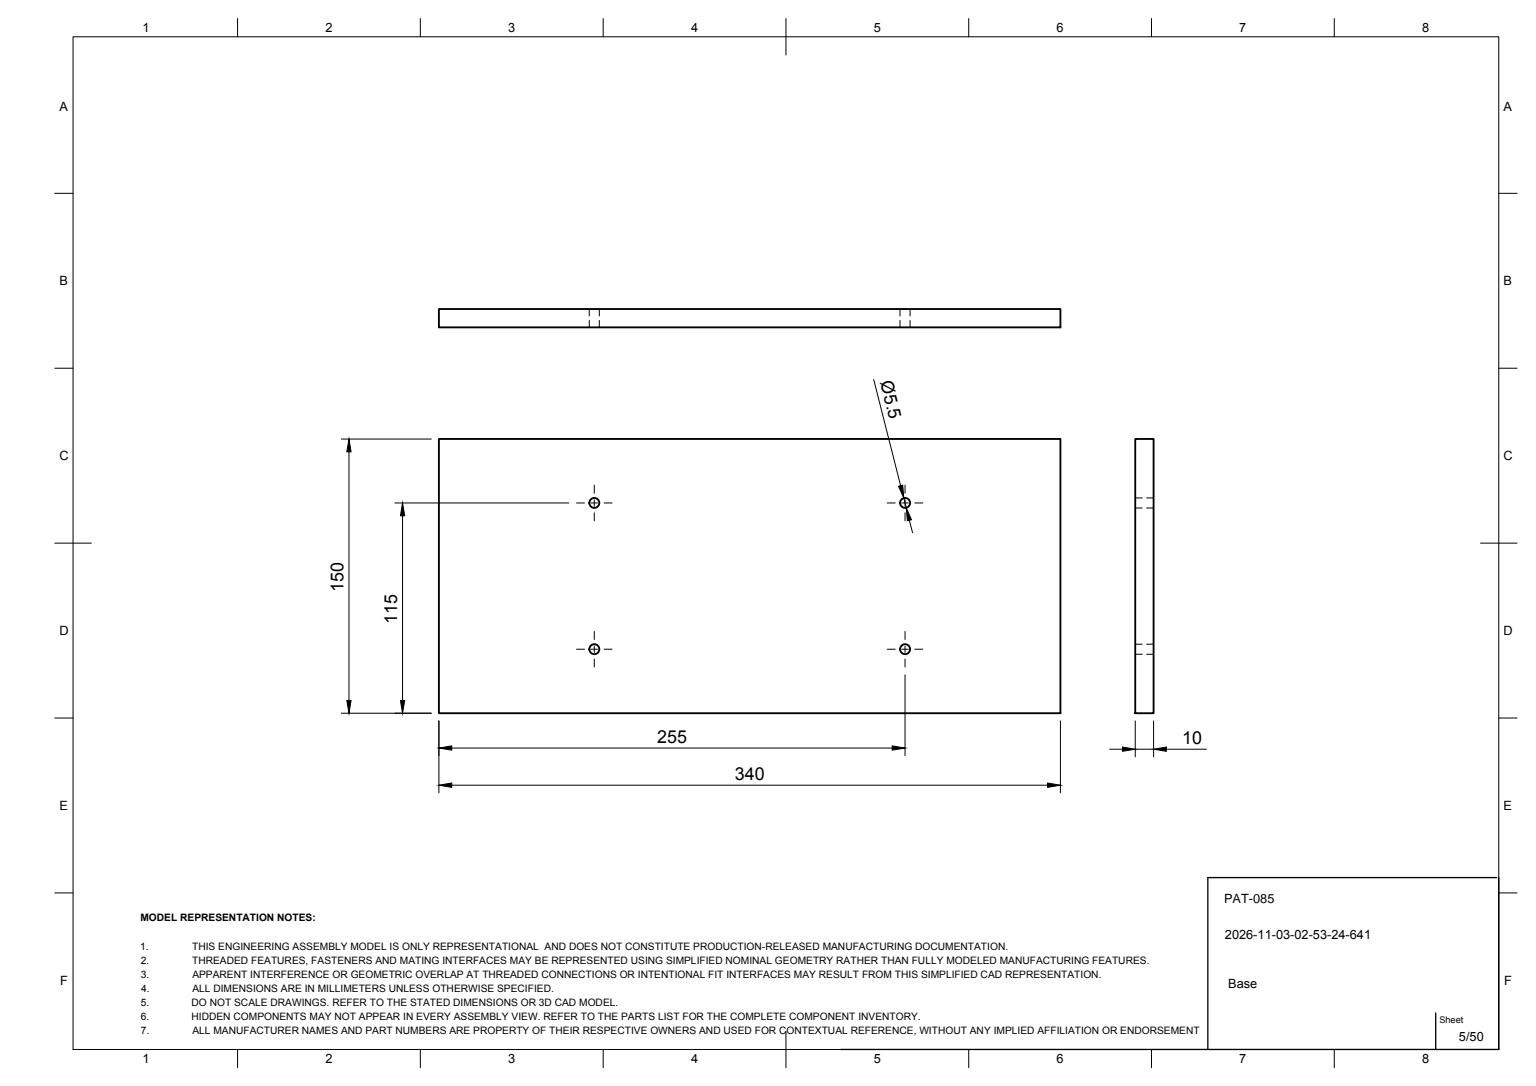
ISO-10303-21;
HEADER;
/* Generated by software containing ST-Developer
 * from STEP Tools, Inc. (www.steptools.com) 
 */

FILE_DESCRIPTION(
/* description */ ('Rack and pinion manual slide'),
/* implementation_level */ '2;1');

FILE_NAME(
/* name */ 'Base.step',
/* time_stamp */ '2026-10-28T03:22:49-07:00',
/* author */ (''),
/* organization */ (''),
/* preprocessor_version */ 'ST-DEVELOPER v20.2',
/* originating_system */ 'Autodesk Translation Framework v15.17.0.0',
/* authorisation */ '');

FILE_SCHEMA (('AUTOMOTIVE_DESIGN { 1 0 10303 214 3 1 1 }'));
ENDSEC;

DATA;
#10=MECHANICAL_DESIGN_GEOMETRIC_PRESENTATION_REPRESENTATION('',(#732),#34851);
#640=SHAPE_REPRESENTATION_RELATIONSHIP('SRR','None',#35075,#686);
#686=ADVANCED_BREP_SHAPE_REPRESENTATION('',(#785),#34800);
#732=STYLED_ITEM('',(#35390),#785);
#785=MANIFOLD_SOLID_BREP('Body1',#13752);
#833=FACE_BOUND('',#2283,.T.);
#834=FACE_BOUND('',#2284,.T.);
#835=FACE_BOUND('',#2285,.T.);
#836=FACE_BOUND('',#2286,.T.);
#837=FACE_BOUND('',#2288,.T.);
#838=FACE_BOUND('',#2289,.T.);
#839=FACE_BOUND('',#2290,.T.);
#840=FACE_BOUND('',#2291,.T.);
#1044=PLANE('',#14332);
#1045=PLANE('',#14333);
#1046=PLANE('',#14334);
#1047=PLANE('',#14335);
#1048=PLANE('',#14336);
#1049=PLANE('',#14337);
#1535=FACE_OUTER_BOUND('',#2274,.T.);
#1536=FACE_OUTER_BOUND('',#2275,.T.);
#1537=FACE_OUTER_BOUND('',#2276,.T.);
#1538=FACE_OUTER_BOUND('',#2277,.T.);
#1539=FACE_OUTER_BOUND('',#2278,.T.);
#1540=FACE_OUTER_BOUND('',#2279,.T.);
#1541=FACE_OUTER_BOUND('',#2280,.T.);
#1542=FACE_OUTER_BOUND('',#2281,.T.);
#1543=FACE_OUTER_BOUND('',#2282,.T.);
#1544=FACE_OUTER_BOUND('',#2287,.T.);
#2274=EDGE_LOOP('',(#9234,#9235,#9236,#9237));
#2275=EDGE_LOOP('',(#9238,#9239,#9240,#9241));
#2276=EDGE_LOOP('',(#9242,#9243,#9244,#9245));
#2277=EDGE_LOOP('',(#9246,#9247,#9248,#9249));
#2278=EDGE_LOOP('',(#9250,#9251,#9252,#9253));
#2279=EDGE_LOOP('',(#9254,#9255,#9256,#9257));
#2280=EDGE_LOOP('',(#9258,#9259,#9260,#9261));
#2281=EDGE_LOOP('',(#9262,#9263,#9264,#9265));
#2282=EDGE_LOOP('',(#9266,#9267,#9268,#9269));
#2283=EDGE_LOOP('',(#9270));
#2284=EDGE_LOOP('',(#9271));
#2285=EDGE_LOOP('',(#9272));
#2286=EDGE_LOOP('',(#9273));
#2287=EDGE_LOOP('',(#9274,#9275,#9276,#9277));
#2288=EDGE_LOOP('',(#9278));
#2289=EDGE_LOOP('',(#9279));
#2290=EDGE_LOOP('',(#9280));
#2291=EDGE_LOOP('',(#9281));
#3224=LINE('',#19464,#4515);
#3225=LINE('',#19470,#4516);
#3226=LINE('',#19476,#4517);
#3227=LINE('',#19482,#4518);
#3228=LINE('',#19487,#4519);
#3229=LINE('',#19489,#4520);
#3230=LINE('',#19491,#4521);
#3231=LINE('',#19492,#4522);
#3232=LINE('',#19495,#4523);
#3233=LINE('',#19497,#4524);
#3234=LINE('',#19498,#4525);
#3235=LINE('',#19501,#4526);
#3236=LINE('',#19503,#4527);
#3237=LINE('',#19504,#4528);
#3238=LINE('',#19506,#4529);
#3239=LINE('',#19507,#4530);
#4515=VECTOR('',#15610,0.274999999999999);
#4516=VECTOR('',#15617,0.274999999999999);
#4517=VECTOR('',#15624,0.275);
#4518=VECTOR('',#15631,0.275);
#4519=VECTOR('',#15636,1.);
#4520=VECTOR('',#15637,1.);
#4521=VECTOR('',#15638,1.);
#4522=VECTOR('',#15639,1.);
#4523=VECTOR('',#15642,1.);
#4524=VECTOR('',#15643,1.);
#4525=VECTOR('',#15644,1.);
#4526=VECTOR('',#15647,1.);
#4527=VECTOR('',#15648,1.);
#4528=VECTOR('',#15649,1.);
#4529=VECTOR('',#15652,1.);
#4530=VECTOR('',#15653,1.);
#5806=CIRCLE('',#14321,0.274999999999999);
#5807=CIRCLE('',#14322,0.274999999999999);
#5808=CIRCLE('',#14324,0.274999999999999);
#5809=CIRCLE('',#14325,0.274999999999999);
#5810=CIRCLE('',#14327,0.275);
#5811=CIRCLE('',#14328,0.275);
#5812=CIRCLE('',#14330,0.275);
#5813=CIRCLE('',#14331,0.275);
#6224=VERTEX_POINT('',#19461);
#6225=VERTEX_POINT('',#19463);
#6226=VERTEX_POINT('',#19467);
#6227=VERTEX_POINT('',#19469);
#6228=VERTEX_POINT('',#19473);
#6229=VERTEX_POINT('',#19475);
#6230=VERTEX_POINT('',#19479);
#6231=VERTEX_POINT('',#19481);
#6232=VERTEX_POINT('',#19485);
#6233=VERTEX_POINT('',#19486);
#6234=VERTEX_POINT('',#19488);
#6235=VERTEX_POINT('',#19490);
#6236=VERTEX_POINT('',#19494);
#6237=VERTEX_POINT('',#19496);
#6238=VERTEX_POINT('',#19500);
#6239=VERTEX_POINT('',#19502);
#7429=EDGE_CURVE('',#6224,#6224,#5806,.T.);
#7430=EDGE_CURVE('',#6224,#6225,#3224,.T.);
#7431=EDGE_CURVE('',#6225,#6225,#5807,.T.);
#7432=EDGE_CURVE('',#6226,#6226,#5808,.T.);
#7433=EDGE_CURVE('',#6226,#6227,#3225,.T.);
#7434=EDGE_CURVE('',#6227,#6227,#5809,.T.);
#7435=EDGE_CURVE('',#6228,#6228,#5810,.T.);
#7436=EDGE_CURVE('',#6228,#6229,#3226,.T.);
#7437=EDGE_CURVE('',#6229,#6229,#5811,.T.);
#7438=EDGE_CURVE('',#6230,#6230,#5812,.T.);
#7439=EDGE_CURVE('',#6230,#6231,#3227,.T.);
#7440=EDGE_CURVE('',#6231,#6231,#5813,.T.);
#7441=EDGE_CURVE('',#6232,#6233,#3228,.T.);
#7442=EDGE_CURVE('',#6233,#6234,#3229,.T.);
#7443=EDGE_CURVE('',#6235,#6234,#3230,.T.);
#7444=EDGE_CURVE('',#6232,#6235,#3231,.T.);
#7445=EDGE_CURVE('',#6236,#6232,#3232,.T.);
#7446=EDGE_CURVE('',#6237,#6235,#3233,.T.);
#7447=EDGE_CURVE('',#6236,#6237,#3234,.T.);
#7448=EDGE_CURVE('',#6238,#6236,#3235,.T.);
#7449=EDGE_CURVE('',#6239,#6237,#3236,.T.);
#7450=EDGE_CURVE('',#6238,#6239,#3237,.T.);
#7451=EDGE_CURVE('',#6233,#6238,#3238,.T.);
#7452=EDGE_CURVE('',#6234,#6239,#3239,.T.);
#9234=ORIENTED_EDGE('',*,*,#7429,.F.);
#9235=ORIENTED_EDGE('',*,*,#7430,.T.);
#9236=ORIENTED_EDGE('',*,*,#7431,.F.);
#9237=ORIENTED_EDGE('',*,*,#7430,.F.);
#9238=ORIENTED_EDGE('',*,*,#7432,.F.);
#9239=ORIENTED_EDGE('',*,*,#7433,.T.);
#9240=ORIENTED_EDGE('',*,*,#7434,.F.);
#9241=ORIENTED_EDGE('',*,*,#7433,.F.);
#9242=ORIENTED_EDGE('',*,*,#7435,.F.);
#9243=ORIENTED_EDGE('',*,*,#7436,.T.);
#9244=ORIENTED_EDGE('',*,*,#7437,.F.);
#9245=ORIENTED_EDGE('',*,*,#7436,.F.);
#9246=ORIENTED_EDGE('',*,*,#7438,.F.);
#9247=ORIENTED_EDGE('',*,*,#7439,.T.);
#9248=ORIENTED_EDGE('',*,*,#7440,.F.);
#9249=ORIENTED_EDGE('',*,*,#7439,.F.);
#9250=ORIENTED_EDGE('',*,*,#7441,.T.);
#9251=ORIENTED_EDGE('',*,*,#7442,.T.);
#9252=ORIENTED_EDGE('',*,*,#7443,.F.);
#9253=ORIENTED_EDGE('',*,*,#7444,.F.);
#9254=ORIENTED_EDGE('',*,*,#7445,.T.);
#9255=ORIENTED_EDGE('',*,*,#7444,.T.);
#9256=ORIENTED_EDGE('',*,*,#7446,.F.);
#9257=ORIENTED_EDGE('',*,*,#7447,.F.);
#9258=ORIENTED_EDGE('',*,*,#7448,.T.);
#9259=ORIENTED_EDGE('',*,*,#7447,.T.);
#9260=ORIENTED_EDGE('',*,*,#7449,.F.);
#9261=ORIENTED_EDGE('',*,*,#7450,.F.);
#9262=ORIENTED_EDGE('',*,*,#7451,.T.);
#9263=ORIENTED_EDGE('',*,*,#7450,.T.);
#9264=ORIENTED_EDGE('',*,*,#7452,.F.);
#9265=ORIENTED_EDGE('',*,*,#7442,.F.);
#9266=ORIENTED_EDGE('',*,*,#7452,.T.);
#9267=ORIENTED_EDGE('',*,*,#7449,.T.);
#9268=ORIENTED_EDGE('',*,*,#7446,.T.);
#9269=ORIENTED_EDGE('',*,*,#7443,.T.);
#9270=ORIENTED_EDGE('',*,*,#7431,.T.);
#9271=ORIENTED_EDGE('',*,*,#7434,.T.);
#9272=ORIENTED_EDGE('',*,*,#7437,.T.);
#9273=ORIENTED_EDGE('',*,*,#7440,.T.);
#9274=ORIENTED_EDGE('',*,*,#7451,.F.);
#9275=ORIENTED_EDGE('',*,*,#7441,.F.);
#9276=ORIENTED_EDGE('',*,*,#7445,.F.);
#9277=ORIENTED_EDGE('',*,*,#7448,.F.);
#9278=ORIENTED_EDGE('',*,*,#7429,.T.);
#9279=ORIENTED_EDGE('',*,*,#7432,.T.);
#9280=ORIENTED_EDGE('',*,*,#7435,.T.);
#9281=ORIENTED_EDGE('',*,*,#7438,.T.);
#12844=CYLINDRICAL_SURFACE('',#14320,0.274999999999999);
#12845=CYLINDRICAL_SURFACE('',#14323,0.274999999999999);
#12846=CYLINDRICAL_SURFACE('',#14326,0.275);
#12847=CYLINDRICAL_SURFACE('',#14329,0.275);
#13013=ADVANCED_FACE('',(#1535),#12844,.F.);
#13014=ADVANCED_FACE('',(#1536),#12845,.F.);
#13015=ADVANCED_FACE('',(#1537),#12846,.F.);
#13016=ADVANCED_FACE('',(#1538),#12847,.F.);
#13017=ADVANCED_FACE('',(#1539),#1044,.T.);
#13018=ADVANCED_FACE('',(#1540),#1045,.T.);
#13019=ADVANCED_FACE('',(#1541),#1046,.T.);
#13020=ADVANCED_FACE('',(#1542),#1047,.T.);
#13021=ADVANCED_FACE('',(#1543,#833,#834,#835,#836),#1048,.T.);
#13022=ADVANCED_FACE('',(#1544,#837,#838,#839,#840),#1049,.F.);
#13752=CLOSED_SHELL('',(#13013,#13014,#13015,#13016,#13017,#13018,#13019,
#13020,#13021,#13022));
#14319=AXIS2_PLACEMENT_3D('',#19459,#15604,#15605);
#14320=AXIS2_PLACEMENT_3D('',#19460,#15606,#15607);
#14321=AXIS2_PLACEMENT_3D('',#19462,#15608,#15609);
#14322=AXIS2_PLACEMENT_3D('',#19465,#15611,#15612);
#14323=AXIS2_PLACEMENT_3D('',#19466,#15613,#15614);
#14324=AXIS2_PLACEMENT_3D('',#19468,#15615,#15616);
#14325=AXIS2_PLACEMENT_3D('',#19471,#15618,#15619);
#14326=AXIS2_PLACEMENT_3D('',#19472,#15620,#15621);
#14327=AXIS2_PLACEMENT_3D('',#19474,#15622,#15623);
#14328=AXIS2_PLACEMENT_3D('',#19477,#15625,#15626);
#14329=AXIS2_PLACEMENT_3D('',#19478,#15627,#15628);
#14330=AXIS2_PLACEMENT_3D('',#19480,#15629,#15630);
#14331=AXIS2_PLACEMENT_3D('',#19483,#15632,#15633);
#14332=AXIS2_PLACEMENT_3D('',#19484,#15634,#15635);
#14333=AXIS2_PLACEMENT_3D('',#19493,#15640,#15641);
#14334=AXIS2_PLACEMENT_3D('',#19499,#15645,#15646);
#14335=AXIS2_PLACEMENT_3D('',#19505,#15650,#15651);
#14336=AXIS2_PLACEMENT_3D('',#19508,#15654,#15655);
#14337=AXIS2_PLACEMENT_3D('',#19509,#15656,#15657);
#15604=DIRECTION('axis',(0.,0.,1.));
#15605=DIRECTION('refdir',(1.,0.,0.));
#15606=DIRECTION('center_axis',(0.,0.,1.));
#15607=DIRECTION('ref_axis',(1.,0.,0.));
#15608=DIRECTION('center_axis',(0.,0.,1.));
#15609=DIRECTION('ref_axis',(1.,0.,0.));
#15610=DIRECTION('',(0.,0.,1.));
#15611=DIRECTION('center_axis',(0.,0.,-1.));
#15612=DIRECTION('ref_axis',(1.,0.,0.));
#15613=DIRECTION('center_axis',(0.,0.,1.));
#15614=DIRECTION('ref_axis',(1.,0.,0.));
#15615=DIRECTION('center_axis',(0.,0.,1.));
#15616=DIRECTION('ref_axis',(1.,0.,0.));
#15617=DIRECTION('',(0.,0.,1.));
#15618=DIRECTION('center_axis',(0.,0.,-1.));
#15619=DIRECTION('ref_axis',(1.,0.,0.));
#15620=DIRECTION('center_axis',(0.,0.,1.));
#15621=DIRECTION('ref_axis',(1.,0.,0.));
#15622=DIRECTION('center_axis',(0.,0.,1.));
#15623=DIRECTION('ref_axis',(1.,0.,0.));
#15624=DIRECTION('',(0.,0.,1.));
#15625=DIRECTION('center_axis',(0.,0.,-1.));
#15626=DIRECTION('ref_axis',(1.,0.,0.));
#15627=DIRECTION('center_axis',(0.,0.,1.));
#15628=DIRECTION('ref_axis',(1.,0.,0.));
#15629=DIRECTION('center_axis',(0.,0.,1.));
#15630=DIRECTION('ref_axis',(1.,0.,0.));
#15631=DIRECTION('',(0.,0.,1.));
#15632=DIRECTION('center_axis',(0.,0.,-1.));
#15633=DIRECTION('ref_axis',(1.,0.,0.));
#15634=DIRECTION('center_axis',(0.,1.,0.));
#15635=DIRECTION('ref_axis',(-1.,0.,0.));
#15636=DIRECTION('',(-1.,0.,0.));
#15637=DIRECTION('',(0.,0.,1.));
#15638=DIRECTION('',(-1.,0.,0.));
#15639=DIRECTION('',(0.,0.,1.));
#15640=DIRECTION('center_axis',(1.,0.,0.));
#15641=DIRECTION('ref_axis',(0.,1.,0.));
#15642=DIRECTION('',(0.,1.,0.));
#15643=DIRECTION('',(0.,1.,0.));
#15644=DIRECTION('',(0.,0.,1.));
#15645=DIRECTION('center_axis',(0.,-1.,0.));
#15646=DIRECTION('ref_axis',(1.,0.,0.));
#15647=DIRECTION('',(1.,0.,0.));
#15648=DIRECTION('',(1.,0.,0.));
#15649=DIRECTION('',(0.,0.,1.));
#15650=DIRECTION('center_axis',(-1.,0.,0.));
#15651=DIRECTION('ref_axis',(0.,-1.,0.));
#15652=DIRECTION('',(0.,-1.,0.));
#15653=DIRECTION('',(0.,-1.,0.));
#15654=DIRECTION('center_axis',(0.,0.,1.));
#15655=DIRECTION('ref_axis',(1.,0.,0.));
#15656=DIRECTION('center_axis',(0.,0.,1.));
#15657=DIRECTION('ref_axis',(1.,0.,0.));
#19459=CARTESIAN_POINT('',(0.,0.,0.));
#19460=CARTESIAN_POINT('Origin',(19.5,4.,-0.1));
#19461=CARTESIAN_POINT('',(19.225,4.,0.));
#19462=CARTESIAN_POINT('Origin',(19.5,4.,0.));
#19463=CARTESIAN_POINT('',(19.225,4.,1.));
#19464=CARTESIAN_POINT('',(19.225,4.,-0.1));
#19465=CARTESIAN_POINT('Origin',(19.5,4.,1.));
#19466=CARTESIAN_POINT('Origin',(19.5,-4.,-0.1));
#19467=CARTESIAN_POINT('',(19.225,-4.,0.));
#19468=CARTESIAN_POINT('Origin',(19.5,-4.,0.));
#19469=CARTESIAN_POINT('',(19.225,-4.,1.));
#19470=CARTESIAN_POINT('',(19.225,-4.,-0.1));
#19471=CARTESIAN_POINT('Origin',(19.5,-4.,1.));
#19472=CARTESIAN_POINT('Origin',(2.5,4.,-0.1));
#19473=CARTESIAN_POINT('',(2.225,4.,0.));
#19474=CARTESIAN_POINT('Origin',(2.5,4.,0.));
#19475=CARTESIAN_POINT('',(2.225,4.,1.));
#19476=CARTESIAN_POINT('',(2.225,4.,-0.1));
#19477=CARTESIAN_POINT('Origin',(2.5,4.,1.));
#19478=CARTESIAN_POINT('Origin',(2.5,-4.,-0.1));
#19479=CARTESIAN_POINT('',(2.225,-4.,0.));
#19480=CARTESIAN_POINT('Origin',(2.5,-4.,0.));
#19481=CARTESIAN_POINT('',(2.225,-4.,1.));
#19482=CARTESIAN_POINT('',(2.225,-4.,-0.1));
#19483=CARTESIAN_POINT('Origin',(2.5,-4.,1.));
#19484=CARTESIAN_POINT('Origin',(28.,7.5,0.));
#19485=CARTESIAN_POINT('',(28.,7.5,0.));
#19486=CARTESIAN_POINT('',(-6.,7.5,0.));
#19487=CARTESIAN_POINT('',(28.,7.5,0.));
#19488=CARTESIAN_POINT('',(-6.,7.5,1.));
#19489=CARTESIAN_POINT('',(-6.,7.5,0.));
#19490=CARTESIAN_POINT('',(28.,7.5,1.));
#19491=CARTESIAN_POINT('',(28.,7.5,1.));
#19492=CARTESIAN_POINT('',(28.,7.5,0.));
#19493=CARTESIAN_POINT('Origin',(28.,-7.5,0.));
#19494=CARTESIAN_POINT('',(28.,-7.5,0.));
#19495=CARTESIAN_POINT('',(28.,-7.5,0.));
#19496=CARTESIAN_POINT('',(28.,-7.5,1.));
#19497=CARTESIAN_POINT('',(28.,-7.5,1.));
#19498=CARTESIAN_POINT('',(28.,-7.5,0.));
#19499=CARTESIAN_POINT('Origin',(-6.,-7.5,0.));
#19500=CARTESIAN_POINT('',(-6.,-7.5,0.));
#19501=CARTESIAN_POINT('',(-6.,-7.5,0.));
#19502=CARTESIAN_POINT('',(-6.,-7.5,1.));
#19503=CARTESIAN_POINT('',(-6.,-7.5,1.));
#19504=CARTESIAN_POINT('',(-6.,-7.5,0.));
#19505=CARTESIAN_POINT('Origin',(-6.,7.5,0.));
#19506=CARTESIAN_POINT('',(-6.,7.5,0.));
#19507=CARTESIAN_POINT('',(-6.,7.5,1.));
#19508=CARTESIAN_POINT('Origin',(11.,0.,1.));
#19509=CARTESIAN_POINT('Origin',(11.,0.,0.));
#34746=UNCERTAINTY_MEASURE_WITH_UNIT(LENGTH_MEASURE(0.001),#34852,
'DISTANCE_ACCURACY_VALUE',
'Maximum model space distance between geometric entities at asserted c
onnectivities');
#34797=UNCERTAINTY_MEASURE_WITH_UNIT(LENGTH_MEASURE(0.001),#34852,
'DISTANCE_ACCURACY_VALUE',
'Maximum model space distance between geometric entities at asserted c
onnectivities');
#34800=(
GEOMETRIC_REPRESENTATION_CONTEXT(3)
GLOBAL_UNCERTAINTY_ASSIGNED_CONTEXT((#34746))
GLOBAL_UNIT_ASSIGNED_CONTEXT((#34852,#34854,#34855))
REPRESENTATION_CONTEXT('','3D')
);
#34851=(
GEOMETRIC_REPRESENTATION_CONTEXT(3)
GLOBAL_UNCERTAINTY_ASSIGNED_CONTEXT((#34797))
GLOBAL_UNIT_ASSIGNED_CONTEXT((#34852,#34854,#34855))
REPRESENTATION_CONTEXT('','3D')
);
#34852=(
LENGTH_UNIT()
NAMED_UNIT(*)
SI_UNIT(.CENTI.,.METRE.)
);
#34854=(
NAMED_UNIT(*)
PLANE_ANGLE_UNIT()
SI_UNIT($,.RADIAN.)
);
#34855=(
NAMED_UNIT(*)
SI_UNIT($,.STERADIAN.)
SOLID_ANGLE_UNIT()
);
#34858=SHAPE_DEFINITION_REPRESENTATION(#34911,#35075);
#34911=PRODUCT_DEFINITION_SHAPE('',$,#35129);
#35075=SHAPE_REPRESENTATION('',(#14319),#34800);
#35126=PRODUCT_DEFINITION_CONTEXT('part definition',#35287,'design');
#35129=PRODUCT_DEFINITION('Base','Base',#35182,#35126);
#35182=PRODUCT_DEFINITION_FORMATION('',$,#35291);
#35287=APPLICATION_CONTEXT(
'Core Data for Automotive Mechanical Design Process');
#35288=PRODUCT_CONTEXT('part definition',#35287,'mechanical');
#35291=PRODUCT('Base','Base','Base',(#35288));
#35384=COLOUR_RGB('Dark Blue',0.08,0.2,0.34);
#35385=FILL_AREA_STYLE_COLOUR('',#35384);
#35386=FILL_AREA_STYLE('',(#35385));
#35387=SURFACE_STYLE_FILL_AREA(#35386);
#35388=SURFACE_SIDE_STYLE('',(#35387));
#35389=SURFACE_STYLE_USAGE(.BOTH.,#35388);
#35390=PRESENTATION_STYLE_ASSIGNMENT((#35389));
ENDSEC;
END-ISO-10303-21;
